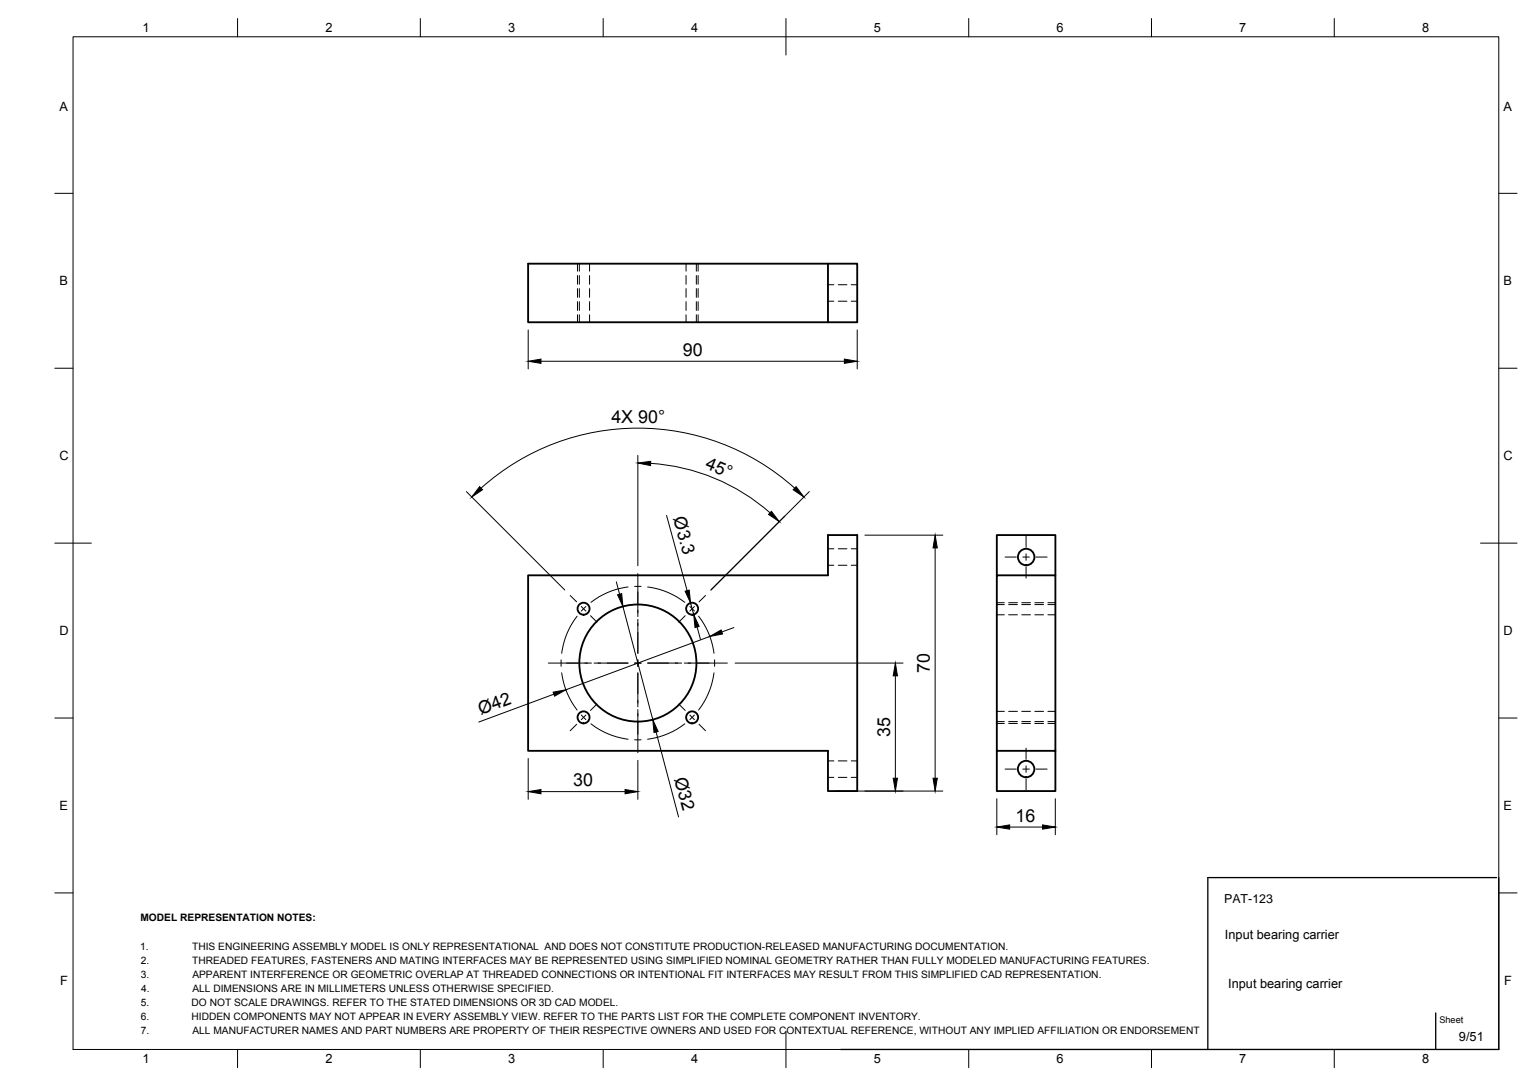
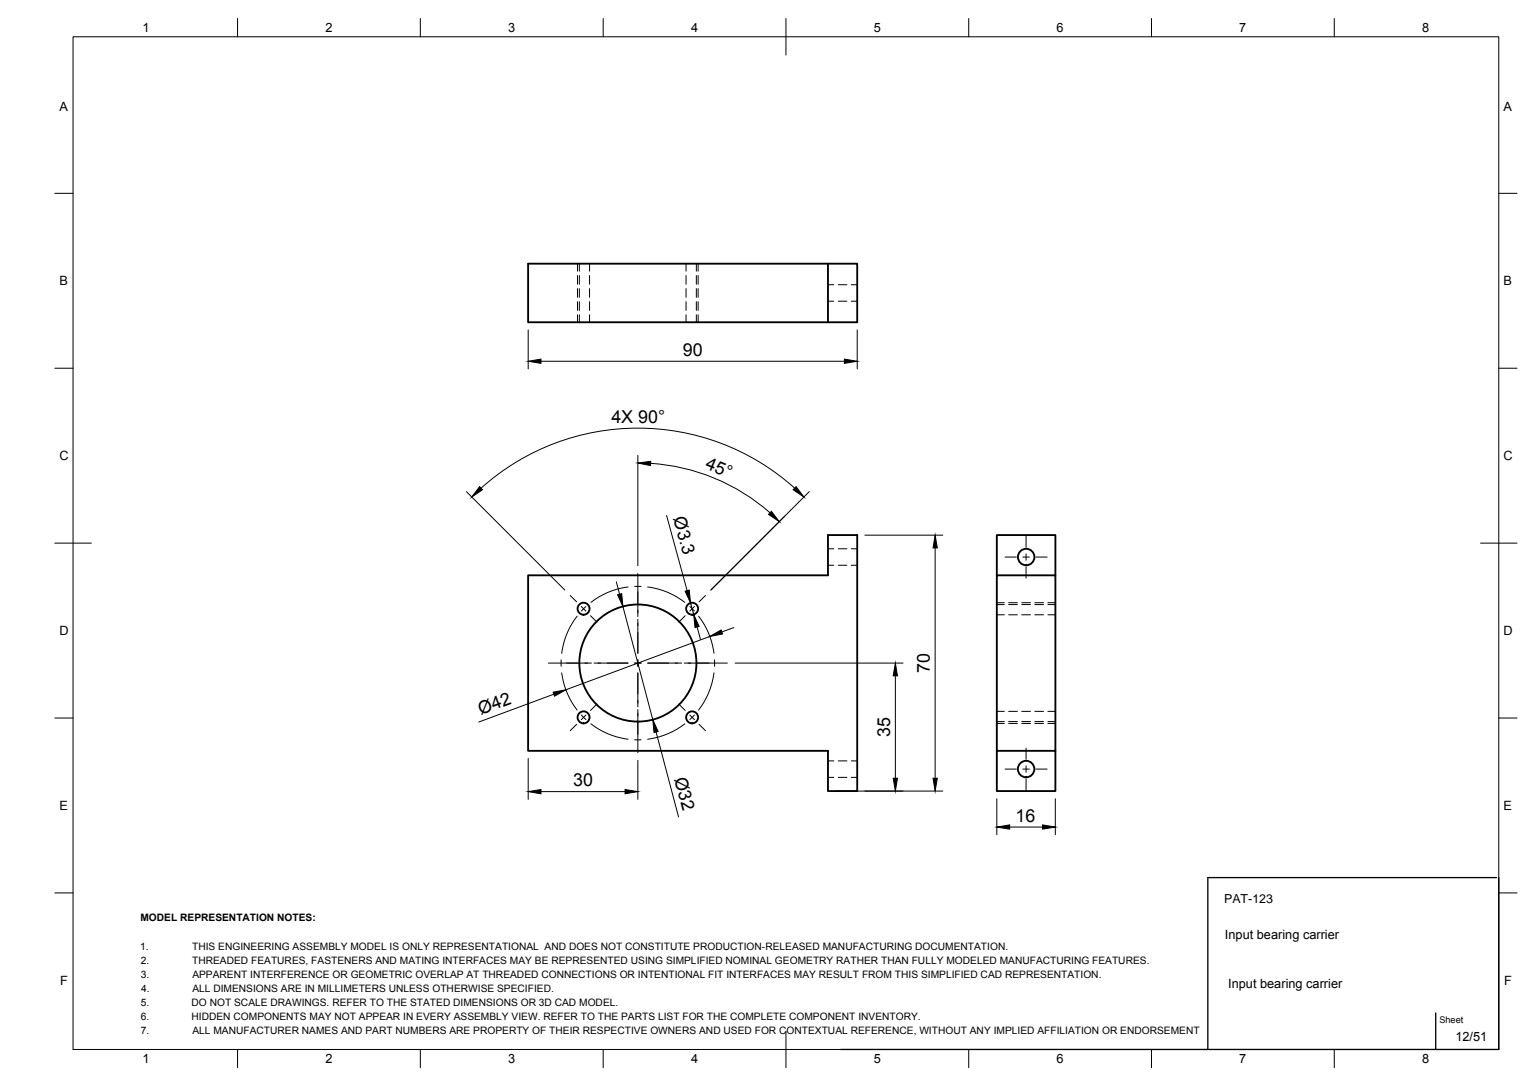
ISO-10303-21;
HEADER;
/* Generated by software containing ST-Developer
 * from STEP Tools, Inc. (www.steptools.com) 
 */

FILE_DESCRIPTION(
/* description */ ('Worm-less right-angle friction wheel drive'),
/* implementation_level */ '2;1');

FILE_NAME(
/* name */ 'Input bearing carrier.step',
/* time_stamp */ '2026-10-28T03:22:36-07:00',
/* author */ (''),
/* organization */ (''),
/* preprocessor_version */ 'ST-DEVELOPER v20.2',
/* originating_system */ 'Autodesk Translation Framework v15.17.0.0',
/* authorisation */ '');

FILE_SCHEMA (('AUTOMOTIVE_DESIGN { 1 0 10303 214 3 1 1 }'));
ENDSEC;

DATA;
#10=MECHANICAL_DESIGN_GEOMETRIC_PRESENTATION_REPRESENTATION('',(#615),#17046);
#521=SHAPE_REPRESENTATION_RELATIONSHIP('SRR','None',#17264,#568);
#568=ADVANCED_BREP_SHAPE_REPRESENTATION('',(#669),#17000);
#615=STYLED_ITEM('',(#17591),#669);
#669=MANIFOLD_SOLID_BREP('Body1',#8170);
#751=FACE_BOUND('',#1772,.T.);
#752=FACE_BOUND('',#1774,.T.);
#753=FACE_BOUND('',#1778,.T.);
#754=FACE_BOUND('',#1779,.T.);
#755=FACE_BOUND('',#1780,.T.);
#756=FACE_BOUND('',#1781,.T.);
#757=FACE_BOUND('',#1782,.T.);
#758=FACE_BOUND('',#1785,.T.);
#759=FACE_BOUND('',#1786,.T.);
#760=FACE_BOUND('',#1787,.T.);
#761=FACE_BOUND('',#1788,.T.);
#762=FACE_BOUND('',#1789,.T.);
#763=FACE_BOUND('',#1793,.T.);
#764=FACE_BOUND('',#1794,.T.);
#984=PLANE('',#8868);
#985=PLANE('',#8869);
#986=PLANE('',#8870);
#987=PLANE('',#8871);
#988=PLANE('',#8872);
#989=PLANE('',#8873);
#990=PLANE('',#8874);
#991=PLANE('',#8875);
#992=PLANE('',#8876);
#993=PLANE('',#8877);
#1262=FACE_OUTER_BOUND('',#1764,.T.);
#1263=FACE_OUTER_BOUND('',#1765,.T.);
#1264=FACE_OUTER_BOUND('',#1766,.T.);
#1265=FACE_OUTER_BOUND('',#1767,.T.);
#1266=FACE_OUTER_BOUND('',#1768,.T.);
#1267=FACE_OUTER_BOUND('',#1769,.T.);
#1268=FACE_OUTER_BOUND('',#1770,.T.);
#1269=FACE_OUTER_BOUND('',#1771,.T.);
#1270=FACE_OUTER_BOUND('',#1773,.T.);
#1271=FACE_OUTER_BOUND('',#1775,.T.);
#1272=FACE_OUTER_BOUND('',#1776,.T.);
#1273=FACE_OUTER_BOUND('',#1777,.T.);
#1274=FACE_OUTER_BOUND('',#1783,.T.);
#1275=FACE_OUTER_BOUND('',#1784,.T.);
#1276=FACE_OUTER_BOUND('',#1790,.T.);
#1277=FACE_OUTER_BOUND('',#1791,.T.);
#1278=FACE_OUTER_BOUND('',#1792,.T.);
#1764=EDGE_LOOP('',(#5810,#5811,#5812,#5813));
#1765=EDGE_LOOP('',(#5814,#5815,#5816,#5817));
#1766=EDGE_LOOP('',(#5818,#5819,#5820,#5821));
#1767=EDGE_LOOP('',(#5822,#5823,#5824,#5825));
#1768=EDGE_LOOP('',(#5826,#5827,#5828,#5829));
#1769=EDGE_LOOP('',(#5830,#5831,#5832,#5833));
#1770=EDGE_LOOP('',(#5834,#5835,#5836,#5837));
#1771=EDGE_LOOP('',(#5838,#5839,#5840,#5841));
#1772=EDGE_LOOP('',(#5842));
#1773=EDGE_LOOP('',(#5843,#5844,#5845,#5846));
#1774=EDGE_LOOP('',(#5847));
#1775=EDGE_LOOP('',(#5848,#5849,#5850,#5851));
#1776=EDGE_LOOP('',(#5852,#5853,#5854,#5855));
#1777=EDGE_LOOP('',(#5856,#5857,#5858,#5859,#5860,#5861,#5862,#5863));
#1778=EDGE_LOOP('',(#5864));
#1779=EDGE_LOOP('',(#5865));
#1780=EDGE_LOOP('',(#5866));
#1781=EDGE_LOOP('',(#5867));
#1782=EDGE_LOOP('',(#5868));
#1783=EDGE_LOOP('',(#5869,#5870,#5871,#5872));
#1784=EDGE_LOOP('',(#5873,#5874,#5875,#5876,#5877,#5878,#5879,#5880));
#1785=EDGE_LOOP('',(#5881));
#1786=EDGE_LOOP('',(#5882));
#1787=EDGE_LOOP('',(#5883));
#1788=EDGE_LOOP('',(#5884));
#1789=EDGE_LOOP('',(#5885));
#1790=EDGE_LOOP('',(#5886,#5887,#5888,#5889));
#1791=EDGE_LOOP('',(#5890,#5891,#5892,#5893));
#1792=EDGE_LOOP('',(#5894,#5895,#5896,#5897));
#1793=EDGE_LOOP('',(#5898));
#1794=EDGE_LOOP('',(#5899));
#2471=LINE('',#12670,#3011);
#2472=LINE('',#12676,#3012);
#2473=LINE('',#12682,#3013);
#2474=LINE('',#12688,#3014);
#2475=LINE('',#12694,#3015);
#2476=LINE('',#12700,#3016);
#2477=LINE('',#12706,#3017);
#2478=LINE('',#12711,#3018);
#2479=LINE('',#12713,#3019);
#2480=LINE('',#12715,#3020);
#2481=LINE('',#12716,#3021);
#2482=LINE('',#12720,#3022);
#2483=LINE('',#12722,#3023);
#2484=LINE('',#12724,#3024);
#2485=LINE('',#12725,#3025);
#2486=LINE('',#12728,#3026);
#2487=LINE('',#12730,#3027);
#2488=LINE('',#12731,#3028);
#2489=LINE('',#12734,#3029);
#2490=LINE('',#12736,#3030);
#2491=LINE('',#12737,#3031);
#2492=LINE('',#12740,#3032);
#2493=LINE('',#12742,#3033);
#2494=LINE('',#12743,#3034);
#2495=LINE('',#12744,#3035);
#2496=LINE('',#12747,#3036);
#2497=LINE('',#12748,#3037);
#2498=LINE('',#12751,#3038);
#2499=LINE('',#12752,#3039);
#2500=LINE('',#12753,#3040);
#2501=LINE('',#12755,#3041);
#3011=VECTOR('',#10081,0.165);
#3012=VECTOR('',#10088,0.165);
#3013=VECTOR('',#10095,0.165);
#3014=VECTOR('',#10102,0.165);
#3015=VECTOR('',#10109,1.6);
#3016=VECTOR('',#10116,0.225);
#3017=VECTOR('',#10123,0.225);
#3018=VECTOR('',#10128,1.);
#3019=VECTOR('',#10129,1.);
#3020=VECTOR('',#10130,1.);
#3021=VECTOR('',#10131,1.);
#3022=VECTOR('',#10134,1.);
#3023=VECTOR('',#10135,1.);
#3024=VECTOR('',#10136,1.);
#3025=VECTOR('',#10137,1.);
#3026=VECTOR('',#10140,1.);
#3027=VECTOR('',#10141,1.);
#3028=VECTOR('',#10142,1.);
#3029=VECTOR('',#10145,1.);
#3030=VECTOR('',#10146,1.);
#3031=VECTOR('',#10147,1.);
#3032=VECTOR('',#10150,1.);
#3033=VECTOR('',#10151,1.);
#3034=VECTOR('',#10152,1.);
#3035=VECTOR('',#10153,1.);
#3036=VECTOR('',#10156,1.);
#3037=VECTOR('',#10157,1.);
#3038=VECTOR('',#10160,1.);
#3039=VECTOR('',#10161,1.);
#3040=VECTOR('',#10162,1.);
#3041=VECTOR('',#10165,1.);
#3501=CIRCLE('',#8848,0.165);
#3502=CIRCLE('',#8849,0.165);
#3503=CIRCLE('',#8851,0.165);
#3504=CIRCLE('',#8852,0.165);
#3505=CIRCLE('',#8854,0.165);
#3506=CIRCLE('',#8855,0.165);
#3507=CIRCLE('',#8857,0.165);
#3508=CIRCLE('',#8858,0.165);
#3509=CIRCLE('',#8860,1.6);
#3510=CIRCLE('',#8861,1.6);
#3511=CIRCLE('',#8863,0.225);
#3512=CIRCLE('',#8864,0.225);
#3513=CIRCLE('',#8866,0.225);
#3514=CIRCLE('',#8867,0.225);
#3961=VERTEX_POINT('',#12667);
#3962=VERTEX_POINT('',#12669);
#3963=VERTEX_POINT('',#12673);
#3964=VERTEX_POINT('',#12675);
#3965=VERTEX_POINT('',#12679);
#3966=VERTEX_POINT('',#12681);
#3967=VERTEX_POINT('',#12685);
#3968=VERTEX_POINT('',#12687);
#3969=VERTEX_POINT('',#12691);
#3970=VERTEX_POINT('',#12693);
#3971=VERTEX_POINT('',#12697);
#3972=VERTEX_POINT('',#12699);
#3973=VERTEX_POINT('',#12703);
#3974=VERTEX_POINT('',#12705);
#3975=VERTEX_POINT('',#12709);
#3976=VERTEX_POINT('',#12710);
#3977=VERTEX_POINT('',#12712);
#3978=VERTEX_POINT('',#12714);
#3979=VERTEX_POINT('',#12718);
#3980=VERTEX_POINT('',#12719);
#3981=VERTEX_POINT('',#12721);
#3982=VERTEX_POINT('',#12723);
#3983=VERTEX_POINT('',#12727);
#3984=VERTEX_POINT('',#12729);
#3985=VERTEX_POINT('',#12733);
#3986=VERTEX_POINT('',#12735);
#3987=VERTEX_POINT('',#12739);
#3988=VERTEX_POINT('',#12741);
#3989=VERTEX_POINT('',#12746);
#3990=VERTEX_POINT('',#12750);
#4674=EDGE_CURVE('',#3961,#3961,#3501,.T.);
#4675=EDGE_CURVE('',#3961,#3962,#2471,.T.);
#4676=EDGE_CURVE('',#3962,#3962,#3502,.T.);
#4677=EDGE_CURVE('',#3963,#3963,#3503,.T.);
#4678=EDGE_CURVE('',#3963,#3964,#2472,.T.);
#4679=EDGE_CURVE('',#3964,#3964,#3504,.T.);
#4680=EDGE_CURVE('',#3965,#3965,#3505,.T.);
#4681=EDGE_CURVE('',#3965,#3966,#2473,.T.);
#4682=EDGE_CURVE('',#3966,#3966,#3506,.T.);
#4683=EDGE_CURVE('',#3967,#3967,#3507,.T.);
#4684=EDGE_CURVE('',#3967,#3968,#2474,.T.);
#4685=EDGE_CURVE('',#3968,#3968,#3508,.T.);
#4686=EDGE_CURVE('',#3969,#3969,#3509,.T.);
#4687=EDGE_CURVE('',#3969,#3970,#2475,.T.);
#4688=EDGE_CURVE('',#3970,#3970,#3510,.T.);
#4689=EDGE_CURVE('',#3971,#3971,#3511,.T.);
#4690=EDGE_CURVE('',#3971,#3972,#2476,.T.);
#4691=EDGE_CURVE('',#3972,#3972,#3512,.T.);
#4692=EDGE_CURVE('',#3973,#3973,#3513,.T.);
#4693=EDGE_CURVE('',#3973,#3974,#2477,.T.);
#4694=EDGE_CURVE('',#3974,#3974,#3514,.T.);
#4695=EDGE_CURVE('',#3975,#3976,#2478,.T.);
#4696=EDGE_CURVE('',#3977,#3975,#2479,.T.);
#4697=EDGE_CURVE('',#3977,#3978,#2480,.T.);
#4698=EDGE_CURVE('',#3976,#3978,#2481,.T.);
#4699=EDGE_CURVE('',#3979,#3980,#2482,.T.);
#4700=EDGE_CURVE('',#3981,#3979,#2483,.T.);
#4701=EDGE_CURVE('',#3982,#3981,#2484,.T.);
#4702=EDGE_CURVE('',#3980,#3982,#2485,.T.);
#4703=EDGE_CURVE('',#3982,#3983,#2486,.T.);
#4704=EDGE_CURVE('',#3984,#3981,#2487,.T.);
#4705=EDGE_CURVE('',#3983,#3984,#2488,.T.);
#4706=EDGE_CURVE('',#3985,#3977,#2489,.T.);
#4707=EDGE_CURVE('',#3985,#3986,#2490,.T.);
#4708=EDGE_CURVE('',#3978,#3986,#2491,.T.);
#4709=EDGE_CURVE('',#3975,#3987,#2492,.T.);
#4710=EDGE_CURVE('',#3988,#3987,#2493,.T.);
#4711=EDGE_CURVE('',#3980,#3988,#2494,.T.);
#4712=EDGE_CURVE('',#3983,#3985,#2495,.T.);
#4713=EDGE_CURVE('',#3976,#3989,#2496,.T.);
#4714=EDGE_CURVE('',#3987,#3989,#2497,.T.);
#4715=EDGE_CURVE('',#3979,#3990,#2498,.T.);
#4716=EDGE_CURVE('',#3989,#3990,#2499,.T.);
#4717=EDGE_CURVE('',#3986,#3984,#2500,.T.);
#4718=EDGE_CURVE('',#3990,#3988,#2501,.T.);
#5810=ORIENTED_EDGE('',*,*,#4674,.F.);
#5811=ORIENTED_EDGE('',*,*,#4675,.T.);
#5812=ORIENTED_EDGE('',*,*,#4676,.F.);
#5813=ORIENTED_EDGE('',*,*,#4675,.F.);
#5814=ORIENTED_EDGE('',*,*,#4677,.F.);
#5815=ORIENTED_EDGE('',*,*,#4678,.T.);
#5816=ORIENTED_EDGE('',*,*,#4679,.F.);
#5817=ORIENTED_EDGE('',*,*,#4678,.F.);
#5818=ORIENTED_EDGE('',*,*,#4680,.F.);
#5819=ORIENTED_EDGE('',*,*,#4681,.T.);
#5820=ORIENTED_EDGE('',*,*,#4682,.F.);
#5821=ORIENTED_EDGE('',*,*,#4681,.F.);
#5822=ORIENTED_EDGE('',*,*,#4683,.F.);
#5823=ORIENTED_EDGE('',*,*,#4684,.T.);
#5824=ORIENTED_EDGE('',*,*,#4685,.F.);
#5825=ORIENTED_EDGE('',*,*,#4684,.F.);
#5826=ORIENTED_EDGE('',*,*,#4686,.F.);
#5827=ORIENTED_EDGE('',*,*,#4687,.T.);
#5828=ORIENTED_EDGE('',*,*,#4688,.F.);
#5829=ORIENTED_EDGE('',*,*,#4687,.F.);
#5830=ORIENTED_EDGE('',*,*,#4689,.F.);
#5831=ORIENTED_EDGE('',*,*,#4690,.T.);
#5832=ORIENTED_EDGE('',*,*,#4691,.F.);
#5833=ORIENTED_EDGE('',*,*,#4690,.F.);
#5834=ORIENTED_EDGE('',*,*,#4692,.F.);
#5835=ORIENTED_EDGE('',*,*,#4693,.T.);
#5836=ORIENTED_EDGE('',*,*,#4694,.F.);
#5837=ORIENTED_EDGE('',*,*,#4693,.F.);
#5838=ORIENTED_EDGE('',*,*,#4695,.F.);
#5839=ORIENTED_EDGE('',*,*,#4696,.F.);
#5840=ORIENTED_EDGE('',*,*,#4697,.T.);
#5841=ORIENTED_EDGE('',*,*,#4698,.F.);
#5842=ORIENTED_EDGE('',*,*,#4694,.T.);
#5843=ORIENTED_EDGE('',*,*,#4699,.F.);
#5844=ORIENTED_EDGE('',*,*,#4700,.F.);
#5845=ORIENTED_EDGE('',*,*,#4701,.F.);
#5846=ORIENTED_EDGE('',*,*,#4702,.F.);
#5847=ORIENTED_EDGE('',*,*,#4691,.T.);
#5848=ORIENTED_EDGE('',*,*,#4703,.F.);
#5849=ORIENTED_EDGE('',*,*,#4701,.T.);
#5850=ORIENTED_EDGE('',*,*,#4704,.F.);
#5851=ORIENTED_EDGE('',*,*,#4705,.F.);
#5852=ORIENTED_EDGE('',*,*,#4706,.F.);
#5853=ORIENTED_EDGE('',*,*,#4707,.T.);
#5854=ORIENTED_EDGE('',*,*,#4708,.F.);
#5855=ORIENTED_EDGE('',*,*,#4697,.F.);
#5856=ORIENTED_EDGE('',*,*,#4709,.T.);
#5857=ORIENTED_EDGE('',*,*,#4710,.F.);
#5858=ORIENTED_EDGE('',*,*,#4711,.F.);
#5859=ORIENTED_EDGE('',*,*,#4702,.T.);
#5860=ORIENTED_EDGE('',*,*,#4703,.T.);
#5861=ORIENTED_EDGE('',*,*,#4712,.T.);
#5862=ORIENTED_EDGE('',*,*,#4706,.T.);
#5863=ORIENTED_EDGE('',*,*,#4696,.T.);
#5864=ORIENTED_EDGE('',*,*,#4686,.T.);
#5865=ORIENTED_EDGE('',*,*,#4683,.T.);
#5866=ORIENTED_EDGE('',*,*,#4680,.T.);
#5867=ORIENTED_EDGE('',*,*,#4677,.T.);
#5868=ORIENTED_EDGE('',*,*,#4674,.T.);
#5869=ORIENTED_EDGE('',*,*,#4695,.T.);
#5870=ORIENTED_EDGE('',*,*,#4713,.T.);
#5871=ORIENTED_EDGE('',*,*,#4714,.F.);
#5872=ORIENTED_EDGE('',*,*,#4709,.F.);
#5873=ORIENTED_EDGE('',*,*,#4715,.T.);
#5874=ORIENTED_EDGE('',*,*,#4716,.F.);
#5875=ORIENTED_EDGE('',*,*,#4713,.F.);
#5876=ORIENTED_EDGE('',*,*,#4698,.T.);
#5877=ORIENTED_EDGE('',*,*,#4708,.T.);
#5878=ORIENTED_EDGE('',*,*,#4717,.T.);
#5879=ORIENTED_EDGE('',*,*,#4704,.T.);
#5880=ORIENTED_EDGE('',*,*,#4700,.T.);
#5881=ORIENTED_EDGE('',*,*,#4688,.T.);
#5882=ORIENTED_EDGE('',*,*,#4685,.T.);
#5883=ORIENTED_EDGE('',*,*,#4682,.T.);
#5884=ORIENTED_EDGE('',*,*,#4679,.T.);
#5885=ORIENTED_EDGE('',*,*,#4676,.T.);
#5886=ORIENTED_EDGE('',*,*,#4699,.T.);
#5887=ORIENTED_EDGE('',*,*,#4711,.T.);
#5888=ORIENTED_EDGE('',*,*,#4718,.F.);
#5889=ORIENTED_EDGE('',*,*,#4715,.F.);
#5890=ORIENTED_EDGE('',*,*,#4718,.T.);
#5891=ORIENTED_EDGE('',*,*,#4710,.T.);
#5892=ORIENTED_EDGE('',*,*,#4714,.T.);
#5893=ORIENTED_EDGE('',*,*,#4716,.T.);
#5894=ORIENTED_EDGE('',*,*,#4717,.F.);
#5895=ORIENTED_EDGE('',*,*,#4707,.F.);
#5896=ORIENTED_EDGE('',*,*,#4712,.F.);
#5897=ORIENTED_EDGE('',*,*,#4705,.T.);
#5898=ORIENTED_EDGE('',*,*,#4689,.T.);
#5899=ORIENTED_EDGE('',*,*,#4692,.T.);
#7552=CYLINDRICAL_SURFACE('',#8847,0.165);
#7553=CYLINDRICAL_SURFACE('',#8850,0.165);
#7554=CYLINDRICAL_SURFACE('',#8853,0.165);
#7555=CYLINDRICAL_SURFACE('',#8856,0.165);
#7556=CYLINDRICAL_SURFACE('',#8859,1.6);
#7557=CYLINDRICAL_SURFACE('',#8862,0.225);
#7558=CYLINDRICAL_SURFACE('',#8865,0.225);
#7754=ADVANCED_FACE('',(#1262),#7552,.F.);
#7755=ADVANCED_FACE('',(#1263),#7553,.F.);
#7756=ADVANCED_FACE('',(#1264),#7554,.F.);
#7757=ADVANCED_FACE('',(#1265),#7555,.F.);
#7758=ADVANCED_FACE('',(#1266),#7556,.F.);
#7759=ADVANCED_FACE('',(#1267),#7557,.F.);
#7760=ADVANCED_FACE('',(#1268),#7558,.F.);
#7761=ADVANCED_FACE('',(#1269,#751),#984,.T.);
#7762=ADVANCED_FACE('',(#1270,#752),#985,.T.);
#7763=ADVANCED_FACE('',(#1271),#986,.T.);
#7764=ADVANCED_FACE('',(#1272),#987,.T.);
#7765=ADVANCED_FACE('',(#1273,#753,#754,#755,#756,#757),#988,.T.);
#7766=ADVANCED_FACE('',(#1274),#989,.T.);
#7767=ADVANCED_FACE('',(#1275,#758,#759,#760,#761,#762),#990,.T.);
#7768=ADVANCED_FACE('',(#1276),#991,.T.);
#7769=ADVANCED_FACE('',(#1277),#992,.T.);
#7770=ADVANCED_FACE('',(#1278,#763,#764),#993,.F.);
#8170=CLOSED_SHELL('',(#7754,#7755,#7756,#7757,#7758,#7759,#7760,#7761,
#7762,#7763,#7764,#7765,#7766,#7767,#7768,#7769,#7770));
#8846=AXIS2_PLACEMENT_3D('',#12665,#10075,#10076);
#8847=AXIS2_PLACEMENT_3D('',#12666,#10077,#10078);
#8848=AXIS2_PLACEMENT_3D('',#12668,#10079,#10080);
#8849=AXIS2_PLACEMENT_3D('',#12671,#10082,#10083);
#8850=AXIS2_PLACEMENT_3D('',#12672,#10084,#10085);
#8851=AXIS2_PLACEMENT_3D('',#12674,#10086,#10087);
#8852=AXIS2_PLACEMENT_3D('',#12677,#10089,#10090);
#8853=AXIS2_PLACEMENT_3D('',#12678,#10091,#10092);
#8854=AXIS2_PLACEMENT_3D('',#12680,#10093,#10094);
#8855=AXIS2_PLACEMENT_3D('',#12683,#10096,#10097);
#8856=AXIS2_PLACEMENT_3D('',#12684,#10098,#10099);
#8857=AXIS2_PLACEMENT_3D('',#12686,#10100,#10101);
#8858=AXIS2_PLACEMENT_3D('',#12689,#10103,#10104);
#8859=AXIS2_PLACEMENT_3D('',#12690,#10105,#10106);
#8860=AXIS2_PLACEMENT_3D('',#12692,#10107,#10108);
#8861=AXIS2_PLACEMENT_3D('',#12695,#10110,#10111);
#8862=AXIS2_PLACEMENT_3D('',#12696,#10112,#10113);
#8863=AXIS2_PLACEMENT_3D('',#12698,#10114,#10115);
#8864=AXIS2_PLACEMENT_3D('',#12701,#10117,#10118);
#8865=AXIS2_PLACEMENT_3D('',#12702,#10119,#10120);
#8866=AXIS2_PLACEMENT_3D('',#12704,#10121,#10122);
#8867=AXIS2_PLACEMENT_3D('',#12707,#10124,#10125);
#8868=AXIS2_PLACEMENT_3D('',#12708,#10126,#10127);
#8869=AXIS2_PLACEMENT_3D('',#12717,#10132,#10133);
#8870=AXIS2_PLACEMENT_3D('',#12726,#10138,#10139);
#8871=AXIS2_PLACEMENT_3D('',#12732,#10143,#10144);
#8872=AXIS2_PLACEMENT_3D('',#12738,#10148,#10149);
#8873=AXIS2_PLACEMENT_3D('',#12745,#10154,#10155);
#8874=AXIS2_PLACEMENT_3D('',#12749,#10158,#10159);
#8875=AXIS2_PLACEMENT_3D('',#12754,#10163,#10164);
#8876=AXIS2_PLACEMENT_3D('',#12756,#10166,#10167);
#8877=AXIS2_PLACEMENT_3D('',#12757,#10168,#10169);
#10075=DIRECTION('axis',(0.,0.,1.));
#10076=DIRECTION('refdir',(1.,0.,0.));
#10077=DIRECTION('center_axis',(0.,1.,0.));
#10078=DIRECTION('ref_axis',(1.,0.,0.));
#10079=DIRECTION('center_axis',(0.,1.,0.));
#10080=DIRECTION('ref_axis',(1.,0.,0.));
#10081=DIRECTION('',(0.,1.,0.));
#10082=DIRECTION('center_axis',(0.,-1.,0.));
#10083=DIRECTION('ref_axis',(1.,0.,0.));
#10084=DIRECTION('center_axis',(0.,1.,0.));
#10085=DIRECTION('ref_axis',(1.,0.,0.));
#10086=DIRECTION('center_axis',(0.,1.,0.));
#10087=DIRECTION('ref_axis',(1.,0.,0.));
#10088=DIRECTION('',(0.,1.,0.));
#10089=DIRECTION('center_axis',(0.,-1.,0.));
#10090=DIRECTION('ref_axis',(1.,0.,0.));
#10091=DIRECTION('center_axis',(0.,1.,0.));
#10092=DIRECTION('ref_axis',(1.,0.,0.));
#10093=DIRECTION('center_axis',(0.,1.,0.));
#10094=DIRECTION('ref_axis',(1.,0.,0.));
#10095=DIRECTION('',(0.,1.,0.));
#10096=DIRECTION('center_axis',(0.,-1.,0.));
#10097=DIRECTION('ref_axis',(1.,0.,0.));
#10098=DIRECTION('center_axis',(0.,1.,0.));
#10099=DIRECTION('ref_axis',(1.,0.,0.));
#10100=DIRECTION('center_axis',(0.,1.,0.));
#10101=DIRECTION('ref_axis',(1.,0.,0.));
#10102=DIRECTION('',(0.,1.,0.));
#10103=DIRECTION('center_axis',(0.,-1.,0.));
#10104=DIRECTION('ref_axis',(1.,0.,0.));
#10105=DIRECTION('center_axis',(0.,1.,0.));
#10106=DIRECTION('ref_axis',(1.,0.,0.));
#10107=DIRECTION('center_axis',(0.,1.,0.));
#10108=DIRECTION('ref_axis',(1.,0.,0.));
#10109=DIRECTION('',(0.,1.,0.));
#10110=DIRECTION('center_axis',(0.,-1.,0.));
#10111=DIRECTION('ref_axis',(1.,0.,0.));
#10112=DIRECTION('center_axis',(0.,0.,1.));
#10113=DIRECTION('ref_axis',(1.,0.,0.));
#10114=DIRECTION('center_axis',(0.,0.,1.));
#10115=DIRECTION('ref_axis',(1.,0.,0.));
#10116=DIRECTION('',(0.,0.,1.));
#10117=DIRECTION('center_axis',(0.,0.,-1.));
#10118=DIRECTION('ref_axis',(1.,0.,0.));
#10119=DIRECTION('center_axis',(0.,0.,1.));
#10120=DIRECTION('ref_axis',(1.,0.,0.));
#10121=DIRECTION('center_axis',(0.,0.,1.));
#10122=DIRECTION('ref_axis',(1.,0.,0.));
#10123=DIRECTION('',(0.,0.,1.));
#10124=DIRECTION('center_axis',(0.,0.,-1.));
#10125=DIRECTION('ref_axis',(1.,0.,0.));
#10126=DIRECTION('center_axis',(0.,0.,1.));
#10127=DIRECTION('ref_axis',(1.,0.,0.));
#10128=DIRECTION('',(0.,1.,0.));
#10129=DIRECTION('',(-1.,0.,0.));
#10130=DIRECTION('',(0.,1.,0.));
#10131=DIRECTION('',(1.,0.,0.));
#10132=DIRECTION('center_axis',(0.,0.,1.));
#10133=DIRECTION('ref_axis',(1.,0.,0.));
#10134=DIRECTION('',(0.,-1.,0.));
#10135=DIRECTION('',(1.,0.,0.));
#10136=DIRECTION('',(0.,1.,0.));
#10137=DIRECTION('',(-1.,0.,0.));
#10138=DIRECTION('center_axis',(-1.,0.,0.));
#10139=DIRECTION('ref_axis',(0.,0.,1.));
#10140=DIRECTION('',(0.,0.,-1.));
#10141=DIRECTION('',(0.,0.,1.));
#10142=DIRECTION('',(0.,1.,0.));
#10143=DIRECTION('center_axis',(1.,0.,0.));
#10144=DIRECTION('ref_axis',(0.,0.,-1.));
#10145=DIRECTION('',(0.,0.,1.));
#10146=DIRECTION('',(0.,1.,0.));
#10147=DIRECTION('',(0.,0.,-1.));
#10148=DIRECTION('center_axis',(0.,-1.,0.));
#10149=DIRECTION('ref_axis',(1.,0.,0.));
#10150=DIRECTION('',(0.,0.,1.));
#10151=DIRECTION('',(1.,0.,0.));
#10152=DIRECTION('',(0.,0.,1.));
#10153=DIRECTION('',(1.,0.,0.));
#10154=DIRECTION('center_axis',(1.,0.,0.));
#10155=DIRECTION('ref_axis',(0.,1.,0.));
#10156=DIRECTION('',(0.,0.,1.));
#10157=DIRECTION('',(0.,1.,0.));
#10158=DIRECTION('center_axis',(0.,1.,0.));
#10159=DIRECTION('ref_axis',(-1.,0.,0.));
#10160=DIRECTION('',(0.,0.,1.));
#10161=DIRECTION('',(-1.,0.,0.));
#10162=DIRECTION('',(-1.,0.,0.));
#10163=DIRECTION('center_axis',(-1.,0.,0.));
#10164=DIRECTION('ref_axis',(0.,-1.,0.));
#10165=DIRECTION('',(0.,-1.,0.));
#10166=DIRECTION('center_axis',(0.,0.,1.));
#10167=DIRECTION('ref_axis',(1.,0.,0.));
#10168=DIRECTION('center_axis',(0.,0.,1.));
#10169=DIRECTION('ref_axis',(1.,0.,0.));
#12665=CARTESIAN_POINT('',(0.,0.,0.));
#12666=CARTESIAN_POINT('Origin',(-1.48492424049175,-7.9,5.51507575950825));
#12667=CARTESIAN_POINT('',(-1.64992424049175,-7.8,5.51507575950825));
#12668=CARTESIAN_POINT('Origin',(-1.48492424049175,-7.8,5.51507575950825));
#12669=CARTESIAN_POINT('',(-1.64992424049175,-6.2,5.51507575950825));
#12670=CARTESIAN_POINT('',(-1.64992424049175,-7.9,5.51507575950825));
#12671=CARTESIAN_POINT('Origin',(-1.48492424049175,-6.2,5.51507575950825));
#12672=CARTESIAN_POINT('Origin',(-1.48492424049175,-7.9,8.48492424049175));
#12673=CARTESIAN_POINT('',(-1.64992424049175,-7.8,8.48492424049175));
#12674=CARTESIAN_POINT('Origin',(-1.48492424049175,-7.8,8.48492424049175));
#12675=CARTESIAN_POINT('',(-1.64992424049175,-6.2,8.48492424049175));
#12676=CARTESIAN_POINT('',(-1.64992424049175,-7.9,8.48492424049175));
#12677=CARTESIAN_POINT('Origin',(-1.48492424049175,-6.2,8.48492424049175));
#12678=CARTESIAN_POINT('Origin',(1.48492424049175,-7.9,8.48492424049175));
#12679=CARTESIAN_POINT('',(1.31992424049175,-7.8,8.48492424049175));
#12680=CARTESIAN_POINT('Origin',(1.48492424049175,-7.8,8.48492424049175));
#12681=CARTESIAN_POINT('',(1.31992424049175,-6.2,8.48492424049175));
#12682=CARTESIAN_POINT('',(1.31992424049175,-7.9,8.48492424049175));
#12683=CARTESIAN_POINT('Origin',(1.48492424049175,-6.2,8.48492424049175));
#12684=CARTESIAN_POINT('Origin',(1.48492424049175,-7.9,5.51507575950825));
#12685=CARTESIAN_POINT('',(1.31992424049175,-7.8,5.51507575950825));
#12686=CARTESIAN_POINT('Origin',(1.48492424049175,-7.8,5.51507575950825));
#12687=CARTESIAN_POINT('',(1.31992424049175,-6.2,5.51507575950825));
#12688=CARTESIAN_POINT('',(1.31992424049175,-7.9,5.51507575950825));
#12689=CARTESIAN_POINT('Origin',(1.48492424049175,-6.2,5.51507575950825));
#12690=CARTESIAN_POINT('Origin',(0.,-7.9,7.));
#12691=CARTESIAN_POINT('',(-1.6,-7.8,7.));
#12692=CARTESIAN_POINT('Origin',(0.,-7.8,7.));
#12693=CARTESIAN_POINT('',(-1.6,-6.2,7.));
#12694=CARTESIAN_POINT('',(-1.6,-7.9,7.));
#12695=CARTESIAN_POINT('Origin',(0.,-6.2,7.));
#12696=CARTESIAN_POINT('Origin',(-2.9,-7.,0.9));
#12697=CARTESIAN_POINT('',(-3.125,-7.,1.));
#12698=CARTESIAN_POINT('Origin',(-2.9,-7.,1.));
#12699=CARTESIAN_POINT('',(-3.125,-7.,1.8));
#12700=CARTESIAN_POINT('',(-3.125,-7.,0.9));
#12701=CARTESIAN_POINT('Origin',(-2.9,-7.,1.8));
#12702=CARTESIAN_POINT('Origin',(2.9,-7.,0.9));
#12703=CARTESIAN_POINT('',(2.675,-7.,1.));
#12704=CARTESIAN_POINT('Origin',(2.9,-7.,1.));
#12705=CARTESIAN_POINT('',(2.675,-7.,1.8));
#12706=CARTESIAN_POINT('',(2.675,-7.,0.9));
#12707=CARTESIAN_POINT('Origin',(2.9,-7.,1.8));
#12708=CARTESIAN_POINT('Origin',(-3.5,-7.8,1.8));
#12709=CARTESIAN_POINT('',(2.4,-7.8,1.8));
#12710=CARTESIAN_POINT('',(2.4,-6.2,1.8));
#12711=CARTESIAN_POINT('',(2.4,-7.8,1.8));
#12712=CARTESIAN_POINT('',(3.5,-7.8,1.8));
#12713=CARTESIAN_POINT('',(3.5,-7.8,1.8));
#12714=CARTESIAN_POINT('',(3.5,-6.2,1.8));
#12715=CARTESIAN_POINT('',(3.5,-7.8,1.8));
#12716=CARTESIAN_POINT('',(3.5,-6.2,1.8));
#12717=CARTESIAN_POINT('Origin',(-3.5,-7.8,1.8));
#12718=CARTESIAN_POINT('',(-2.4,-6.2,1.8));
#12719=CARTESIAN_POINT('',(-2.4,-7.8,1.8));
#12720=CARTESIAN_POINT('',(-2.4,-7.,1.8));
#12721=CARTESIAN_POINT('',(-3.5,-6.2,1.8));
#12722=CARTESIAN_POINT('',(3.5,-6.2,1.8));
#12723=CARTESIAN_POINT('',(-3.5,-7.8,1.8));
#12724=CARTESIAN_POINT('',(-3.5,-7.8,1.8));
#12725=CARTESIAN_POINT('',(3.5,-7.8,1.8));
#12726=CARTESIAN_POINT('Origin',(-3.5,-7.8,1.));
#12727=CARTESIAN_POINT('',(-3.5,-7.8,1.));
#12728=CARTESIAN_POINT('',(-3.5,-7.8,1.8));
#12729=CARTESIAN_POINT('',(-3.5,-6.2,1.));
#12730=CARTESIAN_POINT('',(-3.5,-6.2,1.8));
#12731=CARTESIAN_POINT('',(-3.5,-7.8,1.));
#12732=CARTESIAN_POINT('Origin',(3.5,-7.8,1.8));
#12733=CARTESIAN_POINT('',(3.5,-7.8,1.));
#12734=CARTESIAN_POINT('',(3.5,-7.8,1.));
#12735=CARTESIAN_POINT('',(3.5,-6.2,1.));
#12736=CARTESIAN_POINT('',(3.5,-7.8,1.));
#12737=CARTESIAN_POINT('',(3.5,-6.2,1.));
#12738=CARTESIAN_POINT('Origin',(-2.4,-7.8,1.));
#12739=CARTESIAN_POINT('',(2.4,-7.8,10.));
#12740=CARTESIAN_POINT('',(2.4,-7.8,1.));
#12741=CARTESIAN_POINT('',(-2.4,-7.8,10.));
#12742=CARTESIAN_POINT('',(-2.4,-7.8,10.));
#12743=CARTESIAN_POINT('',(-2.4,-7.8,1.));
#12744=CARTESIAN_POINT('',(-3.5,-7.8,1.));
#12745=CARTESIAN_POINT('Origin',(2.4,-7.8,1.));
#12746=CARTESIAN_POINT('',(2.4,-6.2,10.));
#12747=CARTESIAN_POINT('',(2.4,-6.2,1.));
#12748=CARTESIAN_POINT('',(2.4,-7.8,10.));
#12749=CARTESIAN_POINT('Origin',(2.4,-6.2,1.));
#12750=CARTESIAN_POINT('',(-2.4,-6.2,10.));
#12751=CARTESIAN_POINT('',(-2.4,-6.2,1.));
#12752=CARTESIAN_POINT('',(2.4,-6.2,10.));
#12753=CARTESIAN_POINT('',(-3.5,-6.2,1.));
#12754=CARTESIAN_POINT('Origin',(-2.4,-6.2,1.));
#12755=CARTESIAN_POINT('',(-2.4,-6.2,10.));
#12756=CARTESIAN_POINT('Origin',(0.,-7.,10.));
#12757=CARTESIAN_POINT('Origin',(0.,-7.,1.));
#16947=UNCERTAINTY_MEASURE_WITH_UNIT(LENGTH_MEASURE(0.001),#17047,
'DISTANCE_ACCURACY_VALUE',
'Maximum model space distance between geometric entities at asserted c
onnectivities');
#16993=UNCERTAINTY_MEASURE_WITH_UNIT(LENGTH_MEASURE(0.001),#17047,
'DISTANCE_ACCURACY_VALUE',
'Maximum model space distance between geometric entities at asserted c
onnectivities');
#17000=(
GEOMETRIC_REPRESENTATION_CONTEXT(3)
GLOBAL_UNCERTAINTY_ASSIGNED_CONTEXT((#16947))
GLOBAL_UNIT_ASSIGNED_CONTEXT((#17047,#17049,#17050))
REPRESENTATION_CONTEXT('','3D')
);
#17046=(
GEOMETRIC_REPRESENTATION_CONTEXT(3)
GLOBAL_UNCERTAINTY_ASSIGNED_CONTEXT((#16993))
GLOBAL_UNIT_ASSIGNED_CONTEXT((#17047,#17049,#17050))
REPRESENTATION_CONTEXT('','3D')
);
#17047=(
LENGTH_UNIT()
NAMED_UNIT(*)
SI_UNIT(.CENTI.,.METRE.)
);
#17049=(
NAMED_UNIT(*)
PLANE_ANGLE_UNIT()
SI_UNIT($,.RADIAN.)
);
#17050=(
NAMED_UNIT(*)
SI_UNIT($,.STERADIAN.)
SOLID_ANGLE_UNIT()
);
#17057=SHAPE_DEFINITION_REPRESENTATION(#17109,#17264);
#17109=PRODUCT_DEFINITION_SHAPE('',$,#17317);
#17264=SHAPE_REPRESENTATION('',(#8846),#17000);
#17310=PRODUCT_DEFINITION_CONTEXT('part definition',#17468,'design');
#17317=PRODUCT_DEFINITION('Input bearing carrier',
'Input bearing carrier',#17369,#17310);
#17369=PRODUCT_DEFINITION_FORMATION('',$,#17476);
#17468=APPLICATION_CONTEXT(
'Core Data for Automotive Mechanical Design Process');
#17469=PRODUCT_CONTEXT('part definition',#17468,'mechanical');
#17476=PRODUCT('Input bearing carrier','Input bearing carrier',
'Input bearing carrier',(#17469));
#17585=COLOUR_RGB('Grey',0.48,0.52,0.57);
#17586=FILL_AREA_STYLE_COLOUR('',#17585);
#17587=FILL_AREA_STYLE('',(#17586));
#17588=SURFACE_STYLE_FILL_AREA(#17587);
#17589=SURFACE_SIDE_STYLE('',(#17588));
#17590=SURFACE_STYLE_USAGE(.BOTH.,#17589);
#17591=PRESENTATION_STYLE_ASSIGNMENT((#17590));
ENDSEC;
END-ISO-10303-21;
